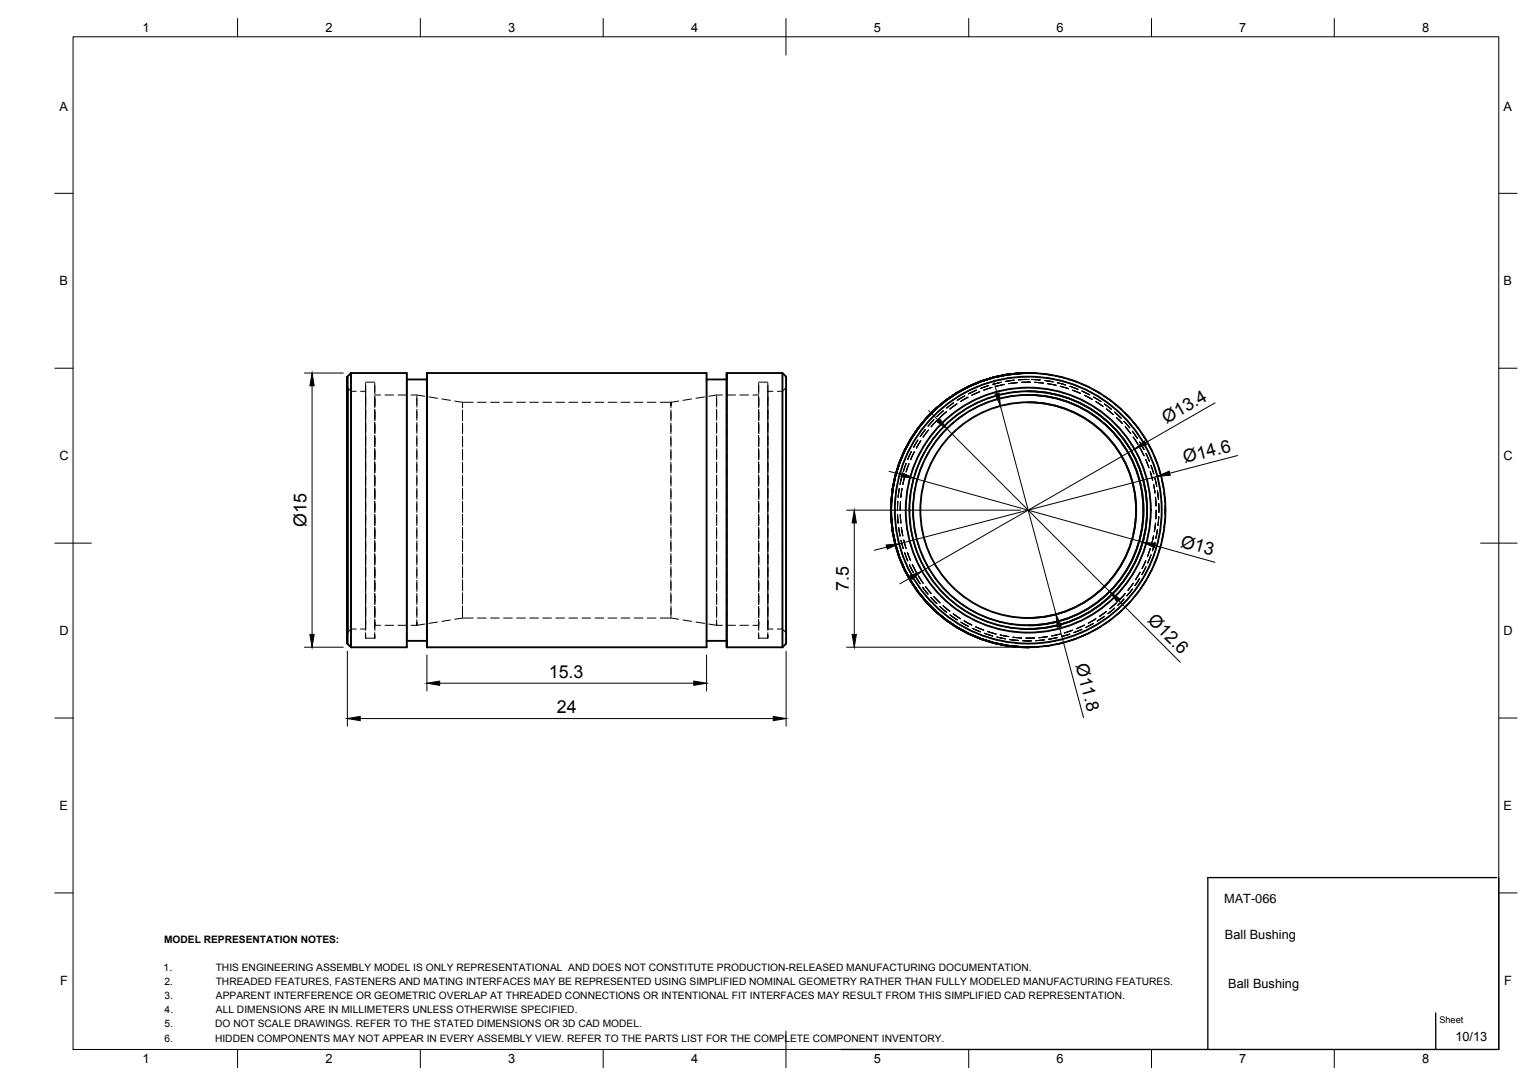
ISO-10303-21;
HEADER;
/* Generated by software containing ST-Developer
 * from STEP Tools, Inc. (www.steptools.com) 
 */

FILE_DESCRIPTION(
/* description */ ('CAx-IF Rec.Pracs.---Representation and Presentation of Product Manufa
cturing Information (PMI)---4.0---2014-10-13'),
/* implementation_level */ '2;1');

FILE_NAME(
/* name */ 'Ball Bushing.step',
/* time_stamp */ '2026-10-24T15:58:00-07:00',
/* author */ (''),
/* organization */ (''),
/* preprocessor_version */ 'ST-DEVELOPER v20.2',
/* originating_system */ 'Autodesk Translation Framework v15.17.0.0',
/* authorisation */ '');

FILE_SCHEMA (('AP242_MANAGED_MODEL_BASED_3D_ENGINEERING_MIM_LF { 1 0 10303 442 2 1 4 }'));
ENDSEC;

DATA;
#10=MECHANICAL_DESIGN_GEOMETRIC_PRESENTATION_REPRESENTATION('',(#134),#8944);
#99=CONICAL_SURFACE('',#5696,0.0066,0.785398163397459);
#100=CONICAL_SURFACE('',#5704,0.0074,0.785398163397448);
#101=CONICAL_SURFACE('',#5709,0.0066,0.785398163397459);
#102=CONICAL_SURFACE('',#5717,0.0074,0.785398163397448);
#103=CONICAL_SURFACE('',#5730,0.0061,0.158655262186402);
#104=CONICAL_SURFACE('',#5734,0.0061,0.158655262186402);
#116=SHAPE_REPRESENTATION_RELATIONSHIP('SRR','None',#8999,#125);
#125=ADVANCED_BREP_SHAPE_REPRESENTATION('',(#143),#8940);
#134=STYLED_ITEM('',(#9054),#143);
#143=MANIFOLD_SOLID_BREP('Body1',#5155);
#220=CYLINDRICAL_SURFACE('',#5702,0.0065);
#221=CYLINDRICAL_SURFACE('',#5707,0.0075);
#222=CYLINDRICAL_SURFACE('',#5715,0.0065);
#223=CYLINDRICAL_SURFACE('',#5720,0.0075);
#224=CYLINDRICAL_SURFACE('',#5724,0.00700000010430813);
#225=CYLINDRICAL_SURFACE('',#5728,0.0063);
#226=CYLINDRICAL_SURFACE('',#5732,0.0059);
#227=CYLINDRICAL_SURFACE('',#5736,0.0063);
#228=CYLINDRICAL_SURFACE('',#5740,0.00700000010430813);
#229=CYLINDRICAL_SURFACE('',#5745,0.00715);
#230=CYLINDRICAL_SURFACE('',#5749,0.0075);
#231=CYLINDRICAL_SURFACE('',#5753,0.00715);
#290=FACE_BOUND('',#854,.T.);
#291=FACE_BOUND('',#860,.T.);
#292=FACE_BOUND('',#865,.T.);
#293=FACE_BOUND('',#868,.T.);
#294=FACE_BOUND('',#875,.T.);
#295=FACE_BOUND('',#878,.T.);
#296=FACE_BOUND('',#880,.T.);
#297=FACE_BOUND('',#883,.T.);
#298=FACE_BOUND('',#886,.T.);
#299=FACE_BOUND('',#889,.T.);
#531=FACE_OUTER_BOUND('',#852,.T.);
#532=FACE_OUTER_BOUND('',#853,.T.);
#533=FACE_OUTER_BOUND('',#855,.T.);
#534=FACE_OUTER_BOUND('',#856,.T.);
#535=FACE_OUTER_BOUND('',#857,.T.);
#536=FACE_OUTER_BOUND('',#858,.T.);
#537=FACE_OUTER_BOUND('',#859,.T.);
#538=FACE_OUTER_BOUND('',#861,.T.);
#539=FACE_OUTER_BOUND('',#862,.T.);
#540=FACE_OUTER_BOUND('',#863,.T.);
#541=FACE_OUTER_BOUND('',#864,.T.);
#542=FACE_OUTER_BOUND('',#866,.T.);
#543=FACE_OUTER_BOUND('',#867,.T.);
#544=FACE_OUTER_BOUND('',#869,.T.);
#545=FACE_OUTER_BOUND('',#870,.T.);
#546=FACE_OUTER_BOUND('',#871,.T.);
#547=FACE_OUTER_BOUND('',#872,.T.);
#548=FACE_OUTER_BOUND('',#873,.T.);
#549=FACE_OUTER_BOUND('',#874,.T.);
#550=FACE_OUTER_BOUND('',#876,.T.);
#551=FACE_OUTER_BOUND('',#877,.T.);
#552=FACE_OUTER_BOUND('',#879,.T.);
#553=FACE_OUTER_BOUND('',#881,.T.);
#554=FACE_OUTER_BOUND('',#882,.T.);
#555=FACE_OUTER_BOUND('',#884,.T.);
#556=FACE_OUTER_BOUND('',#885,.T.);
#557=FACE_OUTER_BOUND('',#887,.T.);
#558=FACE_OUTER_BOUND('',#888,.T.);
#852=EDGE_LOOP('',(#4553,#4554,#4555,#4556,#4557));
#853=EDGE_LOOP('',(#4558));
#854=EDGE_LOOP('',(#4559));
#855=EDGE_LOOP('',(#4560,#4561,#4562,#4563,#4564));
#856=EDGE_LOOP('',(#4565,#4566,#4567,#4568,#4569));
#857=EDGE_LOOP('',(#4570,#4571,#4572,#4573,#4574));
#858=EDGE_LOOP('',(#4575,#4576,#4577,#4578,#4579));
#859=EDGE_LOOP('',(#4580));
#860=EDGE_LOOP('',(#4581));
#861=EDGE_LOOP('',(#4582,#4583,#4584,#4585,#4586));
#862=EDGE_LOOP('',(#4587,#4588,#4589,#4590,#4591));
#863=EDGE_LOOP('',(#4592,#4593,#4594,#4595,#4596));
#864=EDGE_LOOP('',(#4597));
#865=EDGE_LOOP('',(#4598));
#866=EDGE_LOOP('',(#4599,#4600,#4601,#4602));
#867=EDGE_LOOP('',(#4603));
#868=EDGE_LOOP('',(#4604));
#869=EDGE_LOOP('',(#4605,#4606,#4607,#4608));
#870=EDGE_LOOP('',(#4609,#4610,#4611,#4612));
#871=EDGE_LOOP('',(#4613,#4614,#4615,#4616));
#872=EDGE_LOOP('',(#4617,#4618,#4619,#4620));
#873=EDGE_LOOP('',(#4621,#4622,#4623,#4624));
#874=EDGE_LOOP('',(#4625));
#875=EDGE_LOOP('',(#4626));
#876=EDGE_LOOP('',(#4627,#4628,#4629,#4630));
#877=EDGE_LOOP('',(#4631));
#878=EDGE_LOOP('',(#4632));
#879=EDGE_LOOP('',(#4633));
#880=EDGE_LOOP('',(#4634));
#881=EDGE_LOOP('',(#4635,#4636,#4637,#4638));
#882=EDGE_LOOP('',(#4639));
#883=EDGE_LOOP('',(#4640));
#884=EDGE_LOOP('',(#4641,#4642,#4643,#4644));
#885=EDGE_LOOP('',(#4645));
#886=EDGE_LOOP('',(#4646));
#887=EDGE_LOOP('',(#4647,#4648,#4649,#4650));
#888=EDGE_LOOP('',(#4651));
#889=EDGE_LOOP('',(#4652));
#1122=CIRCLE('',#5697,0.00650000000001);
#1123=CIRCLE('',#5698,0.00670000000001);
#1124=CIRCLE('',#5699,0.00650000000001);
#1125=CIRCLE('',#5701,0.00730000000001);
#1126=CIRCLE('',#5703,0.00650000000001);
#1127=CIRCLE('',#5705,0.00750000000001);
#1128=CIRCLE('',#5706,0.00750000000001);
#1129=CIRCLE('',#5708,0.00750000000001);
#1130=CIRCLE('',#5710,0.00650000000001);
#1131=CIRCLE('',#5711,0.00670000000001);
#1132=CIRCLE('',#5712,0.00650000000001);
#1133=CIRCLE('',#5714,0.00730000000001);
#1134=CIRCLE('',#5716,0.00650000000001);
#1135=CIRCLE('',#5718,0.00750000000001);
#1136=CIRCLE('',#5719,0.00750000000001);
#1137=CIRCLE('',#5721,0.00750000000001);
#1138=CIRCLE('',#5723,0.00700000010431813);
#1139=CIRCLE('',#5725,0.00700000010431813);
#1140=CIRCLE('',#5727,0.00630000000001);
#1141=CIRCLE('',#5729,0.00630000000001);
#1142=CIRCLE('',#5731,0.00590000000001);
#1143=CIRCLE('',#5733,0.00590000000001);
#1144=CIRCLE('',#5735,0.00630000000001);
#1145=CIRCLE('',#5737,0.00630000000001);
#1146=CIRCLE('',#5739,0.00700000010431813);
#1147=CIRCLE('',#5741,0.00700000010431813);
#1148=CIRCLE('',#5744,0.00715000000001);
#1149=CIRCLE('',#5746,0.00715000000001);
#1150=CIRCLE('',#5748,0.00750000000001);
#1151=CIRCLE('',#5750,0.00750000000001);
#1152=CIRCLE('',#5752,0.00715000000001);
#1153=CIRCLE('',#5754,0.00715000000001);
#1599=LINE('',#8727,#2054);
#1600=LINE('',#8735,#2055);
#1601=LINE('',#8741,#2056);
#1602=LINE('',#8746,#2057);
#1603=LINE('',#8752,#2058);
#1604=LINE('',#8761,#2059);
#1605=LINE('',#8766,#2060);
#1606=LINE('',#8770,#2061);
#1607=LINE('',#8778,#2062);
#1608=LINE('',#8785,#2063);
#1609=LINE('',#8789,#2064);
#1610=LINE('',#8793,#2065);
#1611=LINE('',#8796,#2066);
#1612=LINE('',#8801,#2067);
#1613=LINE('',#8808,#2068);
#1614=LINE('',#8816,#2069);
#1615=LINE('',#8823,#2070);
#1616=LINE('',#8830,#2071);
#2054=VECTOR('',#7122,0.0066);
#2055=VECTOR('',#7133,0.0065);
#2056=VECTOR('',#7140,0.0074);
#2057=VECTOR('',#7147,0.0075);
#2058=VECTOR('',#7152,0.0066);
#2059=VECTOR('',#7165,0.0065);
#2060=VECTOR('',#7170,0.0074);
#2061=VECTOR('',#7175,0.0075);
#2062=VECTOR('',#7186,0.00700000010430813);
#2063=VECTOR('',#7195,0.0063);
#2064=VECTOR('',#7200,0.0061);
#2065=VECTOR('',#7205,0.0059);
#2066=VECTOR('',#7208,0.0061);
#2067=VECTOR('',#7215,0.0063);
#2068=VECTOR('',#7224,0.00700000010430813);
#2069=VECTOR('',#7235,0.00715);
#2070=VECTOR('',#7244,0.0075);
#2071=VECTOR('',#7253,0.00715);
#2508=VERTEX_POINT('',#8723);
#2509=VERTEX_POINT('',#8724);
#2510=VERTEX_POINT('',#8726);
#2511=VERTEX_POINT('',#8731);
#2512=VERTEX_POINT('',#8734);
#2513=VERTEX_POINT('',#8738);
#2514=VERTEX_POINT('',#8739);
#2515=VERTEX_POINT('',#8744);
#2516=VERTEX_POINT('',#8748);
#2517=VERTEX_POINT('',#8749);
#2518=VERTEX_POINT('',#8751);
#2519=VERTEX_POINT('',#8756);
#2520=VERTEX_POINT('',#8759);
#2521=VERTEX_POINT('',#8763);
#2522=VERTEX_POINT('',#8764);
#2523=VERTEX_POINT('',#8769);
#2524=VERTEX_POINT('',#8773);
#2525=VERTEX_POINT('',#8776);
#2526=VERTEX_POINT('',#8780);
#2527=VERTEX_POINT('',#8783);
#2528=VERTEX_POINT('',#8787);
#2529=VERTEX_POINT('',#8791);
#2530=VERTEX_POINT('',#8795);
#2531=VERTEX_POINT('',#8799);
#2532=VERTEX_POINT('',#8803);
#2533=VERTEX_POINT('',#8806);
#2534=VERTEX_POINT('',#8811);
#2535=VERTEX_POINT('',#8814);
#2536=VERTEX_POINT('',#8818);
#2537=VERTEX_POINT('',#8821);
#2538=VERTEX_POINT('',#8825);
#2539=VERTEX_POINT('',#8828);
#3197=EDGE_CURVE('',#2508,#2509,#1122,.T.);
#3198=EDGE_CURVE('',#2509,#2510,#1599,.T.);
#3199=EDGE_CURVE('',#2510,#2510,#1123,.T.);
#3200=EDGE_CURVE('',#2509,#2508,#1124,.T.);
#3201=EDGE_CURVE('',#2511,#2511,#1125,.T.);
#3202=EDGE_CURVE('',#2508,#2512,#1600,.T.);
#3203=EDGE_CURVE('',#2512,#2512,#1126,.T.);
#3204=EDGE_CURVE('',#2513,#2514,#1127,.T.);
#3205=EDGE_CURVE('',#2514,#2511,#1601,.T.);
#3206=EDGE_CURVE('',#2514,#2513,#1128,.T.);
#3207=EDGE_CURVE('',#2515,#2515,#1129,.T.);
#3208=EDGE_CURVE('',#2515,#2513,#1602,.T.);
#3209=EDGE_CURVE('',#2516,#2517,#1130,.T.);
#3210=EDGE_CURVE('',#2517,#2518,#1603,.T.);
#3211=EDGE_CURVE('',#2518,#2518,#1131,.T.);
#3212=EDGE_CURVE('',#2517,#2516,#1132,.T.);
#3213=EDGE_CURVE('',#2519,#2519,#1133,.T.);
#3214=EDGE_CURVE('',#2520,#2520,#1134,.T.);
#3215=EDGE_CURVE('',#2520,#2516,#1604,.T.);
#3216=EDGE_CURVE('',#2521,#2522,#1135,.T.);
#3217=EDGE_CURVE('',#2522,#2519,#1605,.T.);
#3218=EDGE_CURVE('',#2522,#2521,#1136,.T.);
#3219=EDGE_CURVE('',#2521,#2523,#1606,.T.);
#3220=EDGE_CURVE('',#2523,#2523,#1137,.T.);
#3221=EDGE_CURVE('',#2524,#2524,#1138,.T.);
#3222=EDGE_CURVE('',#2525,#2525,#1139,.T.);
#3223=EDGE_CURVE('',#2525,#2524,#1607,.T.);
#3224=EDGE_CURVE('',#2526,#2526,#1140,.T.);
#3225=EDGE_CURVE('',#2527,#2527,#1141,.T.);
#3226=EDGE_CURVE('',#2527,#2526,#1608,.T.);
#3227=EDGE_CURVE('',#2528,#2528,#1142,.T.);
#3228=EDGE_CURVE('',#2528,#2527,#1609,.T.);
#3229=EDGE_CURVE('',#2529,#2529,#1143,.T.);
#3230=EDGE_CURVE('',#2529,#2528,#1610,.T.);
#3231=EDGE_CURVE('',#2529,#2530,#1611,.T.);
#3232=EDGE_CURVE('',#2530,#2530,#1144,.T.);
#3233=EDGE_CURVE('',#2531,#2531,#1145,.T.);
#3234=EDGE_CURVE('',#2531,#2530,#1612,.T.);
#3235=EDGE_CURVE('',#2532,#2532,#1146,.T.);
#3236=EDGE_CURVE('',#2533,#2533,#1147,.T.);
#3237=EDGE_CURVE('',#2533,#2532,#1613,.T.);
#3238=EDGE_CURVE('',#2534,#2534,#1148,.T.);
#3239=EDGE_CURVE('',#2535,#2535,#1149,.T.);
#3240=EDGE_CURVE('',#2535,#2534,#1614,.T.);
#3241=EDGE_CURVE('',#2536,#2536,#1150,.T.);
#3242=EDGE_CURVE('',#2537,#2537,#1151,.T.);
#3243=EDGE_CURVE('',#2537,#2536,#1615,.T.);
#3244=EDGE_CURVE('',#2538,#2538,#1152,.T.);
#3245=EDGE_CURVE('',#2539,#2539,#1153,.T.);
#3246=EDGE_CURVE('',#2539,#2538,#1616,.T.);
#4553=ORIENTED_EDGE('',*,*,#3197,.T.);
#4554=ORIENTED_EDGE('',*,*,#3198,.T.);
#4555=ORIENTED_EDGE('',*,*,#3199,.T.);
#4556=ORIENTED_EDGE('',*,*,#3198,.F.);
#4557=ORIENTED_EDGE('',*,*,#3200,.T.);
#4558=ORIENTED_EDGE('',*,*,#3201,.F.);
#4559=ORIENTED_EDGE('',*,*,#3199,.F.);
#4560=ORIENTED_EDGE('',*,*,#3197,.F.);
#4561=ORIENTED_EDGE('',*,*,#3202,.T.);
#4562=ORIENTED_EDGE('',*,*,#3203,.T.);
#4563=ORIENTED_EDGE('',*,*,#3202,.F.);
#4564=ORIENTED_EDGE('',*,*,#3200,.F.);
#4565=ORIENTED_EDGE('',*,*,#3204,.T.);
#4566=ORIENTED_EDGE('',*,*,#3205,.T.);
#4567=ORIENTED_EDGE('',*,*,#3201,.T.);
#4568=ORIENTED_EDGE('',*,*,#3205,.F.);
#4569=ORIENTED_EDGE('',*,*,#3206,.T.);
#4570=ORIENTED_EDGE('',*,*,#3207,.F.);
#4571=ORIENTED_EDGE('',*,*,#3208,.T.);
#4572=ORIENTED_EDGE('',*,*,#3206,.F.);
#4573=ORIENTED_EDGE('',*,*,#3204,.F.);
#4574=ORIENTED_EDGE('',*,*,#3208,.F.);
#4575=ORIENTED_EDGE('',*,*,#3209,.T.);
#4576=ORIENTED_EDGE('',*,*,#3210,.T.);
#4577=ORIENTED_EDGE('',*,*,#3211,.T.);
#4578=ORIENTED_EDGE('',*,*,#3210,.F.);
#4579=ORIENTED_EDGE('',*,*,#3212,.T.);
#4580=ORIENTED_EDGE('',*,*,#3213,.F.);
#4581=ORIENTED_EDGE('',*,*,#3211,.F.);
#4582=ORIENTED_EDGE('',*,*,#3214,.F.);
#4583=ORIENTED_EDGE('',*,*,#3215,.T.);
#4584=ORIENTED_EDGE('',*,*,#3212,.F.);
#4585=ORIENTED_EDGE('',*,*,#3209,.F.);
#4586=ORIENTED_EDGE('',*,*,#3215,.F.);
#4587=ORIENTED_EDGE('',*,*,#3216,.T.);
#4588=ORIENTED_EDGE('',*,*,#3217,.T.);
#4589=ORIENTED_EDGE('',*,*,#3213,.T.);
#4590=ORIENTED_EDGE('',*,*,#3217,.F.);
#4591=ORIENTED_EDGE('',*,*,#3218,.T.);
#4592=ORIENTED_EDGE('',*,*,#3216,.F.);
#4593=ORIENTED_EDGE('',*,*,#3219,.T.);
#4594=ORIENTED_EDGE('',*,*,#3220,.T.);
#4595=ORIENTED_EDGE('',*,*,#3219,.F.);
#4596=ORIENTED_EDGE('',*,*,#3218,.F.);
#4597=ORIENTED_EDGE('',*,*,#3221,.F.);
#4598=ORIENTED_EDGE('',*,*,#3214,.T.);
#4599=ORIENTED_EDGE('',*,*,#3222,.F.);
#4600=ORIENTED_EDGE('',*,*,#3223,.T.);
#4601=ORIENTED_EDGE('',*,*,#3221,.T.);
#4602=ORIENTED_EDGE('',*,*,#3223,.F.);
#4603=ORIENTED_EDGE('',*,*,#3222,.T.);
#4604=ORIENTED_EDGE('',*,*,#3224,.F.);
#4605=ORIENTED_EDGE('',*,*,#3225,.F.);
#4606=ORIENTED_EDGE('',*,*,#3226,.T.);
#4607=ORIENTED_EDGE('',*,*,#3224,.T.);
#4608=ORIENTED_EDGE('',*,*,#3226,.F.);
#4609=ORIENTED_EDGE('',*,*,#3227,.F.);
#4610=ORIENTED_EDGE('',*,*,#3228,.T.);
#4611=ORIENTED_EDGE('',*,*,#3225,.T.);
#4612=ORIENTED_EDGE('',*,*,#3228,.F.);
#4613=ORIENTED_EDGE('',*,*,#3229,.F.);
#4614=ORIENTED_EDGE('',*,*,#3230,.T.);
#4615=ORIENTED_EDGE('',*,*,#3227,.T.);
#4616=ORIENTED_EDGE('',*,*,#3230,.F.);
#4617=ORIENTED_EDGE('',*,*,#3229,.T.);
#4618=ORIENTED_EDGE('',*,*,#3231,.T.);
#4619=ORIENTED_EDGE('',*,*,#3232,.F.);
#4620=ORIENTED_EDGE('',*,*,#3231,.F.);
#4621=ORIENTED_EDGE('',*,*,#3233,.F.);
#4622=ORIENTED_EDGE('',*,*,#3234,.T.);
#4623=ORIENTED_EDGE('',*,*,#3232,.T.);
#4624=ORIENTED_EDGE('',*,*,#3234,.F.);
#4625=ORIENTED_EDGE('',*,*,#3235,.F.);
#4626=ORIENTED_EDGE('',*,*,#3233,.T.);
#4627=ORIENTED_EDGE('',*,*,#3236,.F.);
#4628=ORIENTED_EDGE('',*,*,#3237,.T.);
#4629=ORIENTED_EDGE('',*,*,#3235,.T.);
#4630=ORIENTED_EDGE('',*,*,#3237,.F.);
#4631=ORIENTED_EDGE('',*,*,#3236,.T.);
#4632=ORIENTED_EDGE('',*,*,#3203,.F.);
#4633=ORIENTED_EDGE('',*,*,#3207,.T.);
#4634=ORIENTED_EDGE('',*,*,#3238,.F.);
#4635=ORIENTED_EDGE('',*,*,#3239,.F.);
#4636=ORIENTED_EDGE('',*,*,#3240,.T.);
#4637=ORIENTED_EDGE('',*,*,#3238,.T.);
#4638=ORIENTED_EDGE('',*,*,#3240,.F.);
#4639=ORIENTED_EDGE('',*,*,#3241,.F.);
#4640=ORIENTED_EDGE('',*,*,#3239,.T.);
#4641=ORIENTED_EDGE('',*,*,#3242,.F.);
#4642=ORIENTED_EDGE('',*,*,#3243,.T.);
#4643=ORIENTED_EDGE('',*,*,#3241,.T.);
#4644=ORIENTED_EDGE('',*,*,#3243,.F.);
#4645=ORIENTED_EDGE('',*,*,#3242,.T.);
#4646=ORIENTED_EDGE('',*,*,#3244,.F.);
#4647=ORIENTED_EDGE('',*,*,#3245,.F.);
#4648=ORIENTED_EDGE('',*,*,#3246,.T.);
#4649=ORIENTED_EDGE('',*,*,#3244,.T.);
#4650=ORIENTED_EDGE('',*,*,#3246,.F.);
#4651=ORIENTED_EDGE('',*,*,#3220,.F.);
#4652=ORIENTED_EDGE('',*,*,#3245,.T.);
#4863=PLANE('',#5700);
#4864=PLANE('',#5713);
#4865=PLANE('',#5722);
#4866=PLANE('',#5726);
#4867=PLANE('',#5738);
#4868=PLANE('',#5742);
#4869=PLANE('',#5743);
#4870=PLANE('',#5747);
#4871=PLANE('',#5751);
#4872=PLANE('',#5755);
#5104=ADVANCED_FACE('',(#531),#99,.F.);
#5105=ADVANCED_FACE('',(#532,#290),#4863,.T.);
#5106=ADVANCED_FACE('',(#533),#220,.F.);
#5107=ADVANCED_FACE('',(#534),#100,.T.);
#5108=ADVANCED_FACE('',(#535),#221,.T.);
#5109=ADVANCED_FACE('',(#536),#101,.F.);
#5110=ADVANCED_FACE('',(#537,#291),#4864,.T.);
#5111=ADVANCED_FACE('',(#538),#222,.F.);
#5112=ADVANCED_FACE('',(#539),#102,.T.);
#5113=ADVANCED_FACE('',(#540),#223,.T.);
#5114=ADVANCED_FACE('',(#541,#292),#4865,.T.);
#5115=ADVANCED_FACE('',(#542),#224,.F.);
#5116=ADVANCED_FACE('',(#543,#293),#4866,.T.);
#5117=ADVANCED_FACE('',(#544),#225,.F.);
#5118=ADVANCED_FACE('',(#545),#103,.F.);
#5119=ADVANCED_FACE('',(#546),#226,.F.);
#5120=ADVANCED_FACE('',(#547),#104,.F.);
#5121=ADVANCED_FACE('',(#548),#227,.F.);
#5122=ADVANCED_FACE('',(#549,#294),#4867,.T.);
#5123=ADVANCED_FACE('',(#550),#228,.F.);
#5124=ADVANCED_FACE('',(#551,#295),#4868,.T.);
#5125=ADVANCED_FACE('',(#552,#296),#4869,.T.);
#5126=ADVANCED_FACE('',(#553),#229,.T.);
#5127=ADVANCED_FACE('',(#554,#297),#4870,.T.);
#5128=ADVANCED_FACE('',(#555),#230,.T.);
#5129=ADVANCED_FACE('',(#556,#298),#4871,.T.);
#5130=ADVANCED_FACE('',(#557),#231,.T.);
#5131=ADVANCED_FACE('',(#558,#299),#4872,.T.);
#5155=CLOSED_SHELL('',(#5104,#5105,#5106,#5107,#5108,#5109,#5110,#5111,
#5112,#5113,#5114,#5115,#5116,#5117,#5118,#5119,#5120,#5121,#5122,#5123,
#5124,#5125,#5126,#5127,#5128,#5129,#5130,#5131));
#5695=AXIS2_PLACEMENT_3D('',#8721,#7116,#7117);
#5696=AXIS2_PLACEMENT_3D('',#8722,#7118,#7119);
#5697=AXIS2_PLACEMENT_3D('',#8725,#7120,#7121);
#5698=AXIS2_PLACEMENT_3D('',#8728,#7123,#7124);
#5699=AXIS2_PLACEMENT_3D('',#8729,#7125,#7126);
#5700=AXIS2_PLACEMENT_3D('',#8730,#7127,#7128);
#5701=AXIS2_PLACEMENT_3D('',#8732,#7129,#7130);
#5702=AXIS2_PLACEMENT_3D('',#8733,#7131,#7132);
#5703=AXIS2_PLACEMENT_3D('',#8736,#7134,#7135);
#5704=AXIS2_PLACEMENT_3D('',#8737,#7136,#7137);
#5705=AXIS2_PLACEMENT_3D('',#8740,#7138,#7139);
#5706=AXIS2_PLACEMENT_3D('',#8742,#7141,#7142);
#5707=AXIS2_PLACEMENT_3D('',#8743,#7143,#7144);
#5708=AXIS2_PLACEMENT_3D('',#8745,#7145,#7146);
#5709=AXIS2_PLACEMENT_3D('',#8747,#7148,#7149);
#5710=AXIS2_PLACEMENT_3D('',#8750,#7150,#7151);
#5711=AXIS2_PLACEMENT_3D('',#8753,#7153,#7154);
#5712=AXIS2_PLACEMENT_3D('',#8754,#7155,#7156);
#5713=AXIS2_PLACEMENT_3D('',#8755,#7157,#7158);
#5714=AXIS2_PLACEMENT_3D('',#8757,#7159,#7160);
#5715=AXIS2_PLACEMENT_3D('',#8758,#7161,#7162);
#5716=AXIS2_PLACEMENT_3D('',#8760,#7163,#7164);
#5717=AXIS2_PLACEMENT_3D('',#8762,#7166,#7167);
#5718=AXIS2_PLACEMENT_3D('',#8765,#7168,#7169);
#5719=AXIS2_PLACEMENT_3D('',#8767,#7171,#7172);
#5720=AXIS2_PLACEMENT_3D('',#8768,#7173,#7174);
#5721=AXIS2_PLACEMENT_3D('',#8771,#7176,#7177);
#5722=AXIS2_PLACEMENT_3D('',#8772,#7178,#7179);
#5723=AXIS2_PLACEMENT_3D('',#8774,#7180,#7181);
#5724=AXIS2_PLACEMENT_3D('',#8775,#7182,#7183);
#5725=AXIS2_PLACEMENT_3D('',#8777,#7184,#7185);
#5726=AXIS2_PLACEMENT_3D('',#8779,#7187,#7188);
#5727=AXIS2_PLACEMENT_3D('',#8781,#7189,#7190);
#5728=AXIS2_PLACEMENT_3D('',#8782,#7191,#7192);
#5729=AXIS2_PLACEMENT_3D('',#8784,#7193,#7194);
#5730=AXIS2_PLACEMENT_3D('',#8786,#7196,#7197);
#5731=AXIS2_PLACEMENT_3D('',#8788,#7198,#7199);
#5732=AXIS2_PLACEMENT_3D('',#8790,#7201,#7202);
#5733=AXIS2_PLACEMENT_3D('',#8792,#7203,#7204);
#5734=AXIS2_PLACEMENT_3D('',#8794,#7206,#7207);
#5735=AXIS2_PLACEMENT_3D('',#8797,#7209,#7210);
#5736=AXIS2_PLACEMENT_3D('',#8798,#7211,#7212);
#5737=AXIS2_PLACEMENT_3D('',#8800,#7213,#7214);
#5738=AXIS2_PLACEMENT_3D('',#8802,#7216,#7217);
#5739=AXIS2_PLACEMENT_3D('',#8804,#7218,#7219);
#5740=AXIS2_PLACEMENT_3D('',#8805,#7220,#7221);
#5741=AXIS2_PLACEMENT_3D('',#8807,#7222,#7223);
#5742=AXIS2_PLACEMENT_3D('',#8809,#7225,#7226);
#5743=AXIS2_PLACEMENT_3D('',#8810,#7227,#7228);
#5744=AXIS2_PLACEMENT_3D('',#8812,#7229,#7230);
#5745=AXIS2_PLACEMENT_3D('',#8813,#7231,#7232);
#5746=AXIS2_PLACEMENT_3D('',#8815,#7233,#7234);
#5747=AXIS2_PLACEMENT_3D('',#8817,#7236,#7237);
#5748=AXIS2_PLACEMENT_3D('',#8819,#7238,#7239);
#5749=AXIS2_PLACEMENT_3D('',#8820,#7240,#7241);
#5750=AXIS2_PLACEMENT_3D('',#8822,#7242,#7243);
#5751=AXIS2_PLACEMENT_3D('',#8824,#7245,#7246);
#5752=AXIS2_PLACEMENT_3D('',#8826,#7247,#7248);
#5753=AXIS2_PLACEMENT_3D('',#8827,#7249,#7250);
#5754=AXIS2_PLACEMENT_3D('',#8829,#7251,#7252);
#5755=AXIS2_PLACEMENT_3D('',#8831,#7254,#7255);
#7116=DIRECTION('axis',(0.,0.,1.));
#7117=DIRECTION('refdir',(1.,0.,0.));
#7118=DIRECTION('center_axis',(0.,-1.,0.));
#7119=DIRECTION('ref_axis',(0.,0.,-1.));
#7120=DIRECTION('center_axis',(0.,1.,0.));
#7121=DIRECTION('ref_axis',(0.,0.,-1.));
#7122=DIRECTION('',(-8.65956056235503E-17,-0.70710678118654,0.707106781186555));
#7123=DIRECTION('center_axis',(0.,-1.,0.));
#7124=DIRECTION('ref_axis',(0.,0.,-1.));
#7125=DIRECTION('center_axis',(0.,1.,0.));
#7126=DIRECTION('ref_axis',(0.,0.,-1.));
#7127=DIRECTION('center_axis',(0.,-1.,0.));
#7128=DIRECTION('ref_axis',(0.,0.,-1.));
#7129=DIRECTION('center_axis',(0.,1.,0.));
#7130=DIRECTION('ref_axis',(0.,0.,-1.));
#7131=DIRECTION('center_axis',(0.,1.,0.));
#7132=DIRECTION('ref_axis',(0.,0.,1.));
#7133=DIRECTION('',(0.,1.,0.));
#7134=DIRECTION('center_axis',(0.,1.,0.));
#7135=DIRECTION('ref_axis',(1.,0.,0.));
#7136=DIRECTION('center_axis',(0.,1.,0.));
#7137=DIRECTION('ref_axis',(0.,0.,-1.));
#7138=DIRECTION('center_axis',(0.,-1.,0.));
#7139=DIRECTION('ref_axis',(0.,0.,-1.));
#7140=DIRECTION('',(-8.65956056235493E-17,-0.707106781186548,-0.707106781186547));
#7141=DIRECTION('center_axis',(0.,-1.,0.));
#7142=DIRECTION('ref_axis',(0.,0.,-1.));
#7143=DIRECTION('center_axis',(0.,1.,0.));
#7144=DIRECTION('ref_axis',(0.,0.,1.));
#7145=DIRECTION('center_axis',(0.,1.,0.));
#7146=DIRECTION('ref_axis',(1.,0.,0.));
#7147=DIRECTION('',(0.,-1.,0.));
#7148=DIRECTION('center_axis',(0.,1.,0.));
#7149=DIRECTION('ref_axis',(0.,0.,-1.));
#7150=DIRECTION('center_axis',(0.,-1.,0.));
#7151=DIRECTION('ref_axis',(0.,0.,-1.));
#7152=DIRECTION('',(8.65956056235503E-17,0.70710678118654,0.707106781186555));
#7153=DIRECTION('center_axis',(0.,1.,0.));
#7154=DIRECTION('ref_axis',(0.,0.,-1.));
#7155=DIRECTION('center_axis',(0.,-1.,0.));
#7156=DIRECTION('ref_axis',(0.,0.,-1.));
#7157=DIRECTION('center_axis',(0.,1.,0.));
#7158=DIRECTION('ref_axis',(1.,0.,0.));
#7159=DIRECTION('center_axis',(0.,-1.,0.));
#7160=DIRECTION('ref_axis',(0.,0.,-1.));
#7161=DIRECTION('center_axis',(0.,1.,0.));
#7162=DIRECTION('ref_axis',(0.,0.,1.));
#7163=DIRECTION('center_axis',(0.,1.,0.));
#7164=DIRECTION('ref_axis',(1.,0.,0.));
#7165=DIRECTION('',(0.,1.,0.));
#7166=DIRECTION('center_axis',(0.,-1.,0.));
#7167=DIRECTION('ref_axis',(0.,0.,-1.));
#7168=DIRECTION('center_axis',(0.,1.,0.));
#7169=DIRECTION('ref_axis',(0.,0.,-1.));
#7170=DIRECTION('',(8.65956056235493E-17,0.707106781186548,-0.707106781186547));
#7171=DIRECTION('center_axis',(0.,1.,0.));
#7172=DIRECTION('ref_axis',(0.,0.,-1.));
#7173=DIRECTION('center_axis',(0.,1.,0.));
#7174=DIRECTION('ref_axis',(0.,0.,1.));
#7175=DIRECTION('',(0.,-1.,0.));
#7176=DIRECTION('center_axis',(0.,1.,0.));
#7177=DIRECTION('ref_axis',(1.,0.,0.));
#7178=DIRECTION('center_axis',(0.,-1.,0.));
#7179=DIRECTION('ref_axis',(0.,0.,-1.));
#7180=DIRECTION('center_axis',(0.,1.,0.));
#7181=DIRECTION('ref_axis',(1.,0.,0.));
#7182=DIRECTION('center_axis',(0.,1.,0.));
#7183=DIRECTION('ref_axis',(0.,0.,1.));
#7184=DIRECTION('center_axis',(0.,1.,0.));
#7185=DIRECTION('ref_axis',(1.,0.,0.));
#7186=DIRECTION('',(0.,1.,0.));
#7187=DIRECTION('center_axis',(0.,1.,0.));
#7188=DIRECTION('ref_axis',(1.,0.,0.));
#7189=DIRECTION('center_axis',(0.,1.,0.));
#7190=DIRECTION('ref_axis',(1.,0.,0.));
#7191=DIRECTION('center_axis',(0.,1.,0.));
#7192=DIRECTION('ref_axis',(0.,0.,1.));
#7193=DIRECTION('center_axis',(0.,1.,0.));
#7194=DIRECTION('ref_axis',(1.,0.,0.));
#7195=DIRECTION('',(0.,1.,0.));
#7196=DIRECTION('center_axis',(0.,1.,0.));
#7197=DIRECTION('ref_axis',(0.,0.,1.));
#7198=DIRECTION('center_axis',(0.,1.,0.));
#7199=DIRECTION('ref_axis',(1.,0.,0.));
#7200=DIRECTION('',(-1.93482561475974E-17,0.987440631916705,-0.157990501106673));
#7201=DIRECTION('center_axis',(0.,1.,0.));
#7202=DIRECTION('ref_axis',(0.,0.,1.));
#7203=DIRECTION('center_axis',(0.,1.,0.));
#7204=DIRECTION('ref_axis',(1.,0.,0.));
#7205=DIRECTION('',(0.,1.,0.));
#7206=DIRECTION('center_axis',(0.,-1.,0.));
#7207=DIRECTION('ref_axis',(0.,0.,1.));
#7208=DIRECTION('',(1.93482561475974E-17,-0.987440631916705,-0.157990501106673));
#7209=DIRECTION('center_axis',(0.,1.,0.));
#7210=DIRECTION('ref_axis',(1.,0.,0.));
#7211=DIRECTION('center_axis',(0.,1.,0.));
#7212=DIRECTION('ref_axis',(0.,0.,1.));
#7213=DIRECTION('center_axis',(0.,1.,0.));
#7214=DIRECTION('ref_axis',(1.,0.,0.));
#7215=DIRECTION('',(0.,1.,0.));
#7216=DIRECTION('center_axis',(0.,-1.,0.));
#7217=DIRECTION('ref_axis',(0.,0.,-1.));
#7218=DIRECTION('center_axis',(0.,1.,0.));
#7219=DIRECTION('ref_axis',(1.,0.,0.));
#7220=DIRECTION('center_axis',(0.,1.,0.));
#7221=DIRECTION('ref_axis',(0.,0.,1.));
#7222=DIRECTION('center_axis',(0.,1.,0.));
#7223=DIRECTION('ref_axis',(1.,0.,0.));
#7224=DIRECTION('',(0.,1.,0.));
#7225=DIRECTION('center_axis',(0.,1.,0.));
#7226=DIRECTION('ref_axis',(1.,0.,0.));
#7227=DIRECTION('center_axis',(0.,1.,0.));
#7228=DIRECTION('ref_axis',(1.,0.,0.));
#7229=DIRECTION('center_axis',(0.,1.,0.));
#7230=DIRECTION('ref_axis',(1.,0.,0.));
#7231=DIRECTION('center_axis',(0.,1.,0.));
#7232=DIRECTION('ref_axis',(0.,0.,1.));
#7233=DIRECTION('center_axis',(0.,1.,0.));
#7234=DIRECTION('ref_axis',(1.,0.,0.));
#7235=DIRECTION('',(0.,-1.,0.));
#7236=DIRECTION('center_axis',(0.,-1.,0.));
#7237=DIRECTION('ref_axis',(0.,0.,-1.));
#7238=DIRECTION('center_axis',(0.,1.,0.));
#7239=DIRECTION('ref_axis',(1.,0.,0.));
#7240=DIRECTION('center_axis',(0.,1.,0.));
#7241=DIRECTION('ref_axis',(0.,0.,1.));
#7242=DIRECTION('center_axis',(0.,1.,0.));
#7243=DIRECTION('ref_axis',(1.,0.,0.));
#7244=DIRECTION('',(0.,-1.,0.));
#7245=DIRECTION('center_axis',(0.,1.,0.));
#7246=DIRECTION('ref_axis',(1.,0.,0.));
#7247=DIRECTION('center_axis',(0.,1.,0.));
#7248=DIRECTION('ref_axis',(1.,0.,0.));
#7249=DIRECTION('center_axis',(0.,1.,0.));
#7250=DIRECTION('ref_axis',(0.,0.,1.));
#7251=DIRECTION('center_axis',(0.,1.,0.));
#7252=DIRECTION('ref_axis',(1.,0.,0.));
#7253=DIRECTION('',(0.,-1.,0.));
#7254=DIRECTION('center_axis',(0.,-1.,0.));
#7255=DIRECTION('ref_axis',(0.,0.,-1.));
#8721=CARTESIAN_POINT('',(0.,0.,0.));
#8722=CARTESIAN_POINT('Origin',(0.,-0.0119,0.));
#8723=CARTESIAN_POINT('',(0.,-0.01180000000001,-0.00650000000001));
#8724=CARTESIAN_POINT('',(-7.96020419447004E-19,-0.01180000000001,0.00650000000001));
#8725=CARTESIAN_POINT('Origin',(0.,-0.01180000000001,0.));
#8726=CARTESIAN_POINT('',(-8.20513355429951E-19,-0.01200000000001,0.00670000000001));
#8727=CARTESIAN_POINT('',(-8.08266887437253E-19,-0.0119,0.0066));
#8728=CARTESIAN_POINT('Origin',(0.,-0.01200000000001,0.));
#8729=CARTESIAN_POINT('Origin',(0.,-0.01180000000001,0.));
#8730=CARTESIAN_POINT('Origin',(0.,-0.012,0.0075));
#8731=CARTESIAN_POINT('',(8.93992163377568E-19,-0.012,0.0073));
#8732=CARTESIAN_POINT('Origin',(0.,-0.01200000000001,0.));
#8733=CARTESIAN_POINT('Origin',(0.,-0.0115000000819564,0.));
#8734=CARTESIAN_POINT('',(-7.9602041944578E-19,-0.0110000001639228,-0.0065));
#8735=CARTESIAN_POINT('',(-7.9602041944578E-19,-0.0115000000819564,-0.0065));
#8736=CARTESIAN_POINT('Origin',(0.,-0.0110000001639228,0.));
#8737=CARTESIAN_POINT('Origin',(0.,-0.0119,0.));
#8738=CARTESIAN_POINT('',(0.,-0.01180000000001,-0.00750000000001));
#8739=CARTESIAN_POINT('',(9.18485099360515E-19,-0.0118,0.0075));
#8740=CARTESIAN_POINT('Origin',(0.,-0.01180000000001,0.));
#8741=CARTESIAN_POINT('',(9.06238631369041E-19,-0.0119,0.0074));
#8742=CARTESIAN_POINT('Origin',(0.,-0.01180000000001,0.));
#8743=CARTESIAN_POINT('Origin',(0.,-0.010375,0.));
#8744=CARTESIAN_POINT('',(-9.18485099360515E-19,-0.00875000000001,-0.0075));
#8745=CARTESIAN_POINT('Origin',(0.,-0.00875000000001,0.));
#8746=CARTESIAN_POINT('',(-9.18485099360515E-19,-0.010375,-0.0075));
#8747=CARTESIAN_POINT('Origin',(0.,0.0119,0.));
#8748=CARTESIAN_POINT('',(0.,0.01180000000001,-0.00650000000001));
#8749=CARTESIAN_POINT('',(7.96020419447004E-19,0.01180000000001,0.00650000000001));
#8750=CARTESIAN_POINT('Origin',(0.,0.01180000000001,0.));
#8751=CARTESIAN_POINT('',(8.20513355429951E-19,0.01200000000001,0.00670000000001));
#8752=CARTESIAN_POINT('',(8.08266887437253E-19,0.0119,0.0066));
#8753=CARTESIAN_POINT('Origin',(0.,0.01200000000001,0.));
#8754=CARTESIAN_POINT('Origin',(0.,0.01180000000001,0.));
#8755=CARTESIAN_POINT('Origin',(0.,0.012,0.0065));
#8756=CARTESIAN_POINT('',(-8.93992163377568E-19,0.012,0.0073));
#8757=CARTESIAN_POINT('Origin',(0.,0.01200000000001,0.));
#8758=CARTESIAN_POINT('Origin',(0.,0.0115000000819564,0.));
#8759=CARTESIAN_POINT('',(-7.9602041944578E-19,0.0110000001639228,-0.0065));
#8760=CARTESIAN_POINT('Origin',(0.,0.0110000001639228,0.));
#8761=CARTESIAN_POINT('',(-7.9602041944578E-19,0.0115000000819564,-0.0065));
#8762=CARTESIAN_POINT('Origin',(0.,0.0119,0.));
#8763=CARTESIAN_POINT('',(0.,0.01180000000001,-0.00750000000001));
#8764=CARTESIAN_POINT('',(-9.18485099360515E-19,0.0118,0.0075));
#8765=CARTESIAN_POINT('Origin',(0.,0.01180000000001,0.));
#8766=CARTESIAN_POINT('',(-9.06238631369041E-19,0.0119,0.0074));
#8767=CARTESIAN_POINT('Origin',(0.,0.01180000000001,0.));
#8768=CARTESIAN_POINT('Origin',(0.,0.010375,0.));
#8769=CARTESIAN_POINT('',(-9.18485099360515E-19,0.00875000000001,-0.0075));
#8770=CARTESIAN_POINT('',(-9.18485099360515E-19,0.010375,-0.0075));
#8771=CARTESIAN_POINT('Origin',(0.,0.00875000000001,0.));
#8772=CARTESIAN_POINT('Origin',(0.,0.0110000001639128,0.00700000010430813));
#8773=CARTESIAN_POINT('',(-8.57252772177209E-19,0.0110000001639228,-0.00700000010430813));
#8774=CARTESIAN_POINT('Origin',(0.,0.0110000001639228,0.));
#8775=CARTESIAN_POINT('Origin',(0.,0.0107500001601875,0.));
#8776=CARTESIAN_POINT('',(-8.57252772177209E-19,0.0105000001564722,-0.00700000010430813));
#8777=CARTESIAN_POINT('Origin',(0.,0.0105000001564722,0.));
#8778=CARTESIAN_POINT('',(-8.57252772177209E-19,0.0107500001601875,-0.00700000010430813));
#8779=CARTESIAN_POINT('Origin',(0.,0.0105000001564622,0.0063));
#8780=CARTESIAN_POINT('',(-7.71527483462833E-19,0.0105000001564722,-0.0063));
#8781=CARTESIAN_POINT('Origin',(0.,0.0105000001564722,0.));
#8782=CARTESIAN_POINT('Origin',(0.,0.0093500000782311,0.));
#8783=CARTESIAN_POINT('',(-7.71527483462833E-19,0.00820000000001,-0.0063));
#8784=CARTESIAN_POINT('Origin',(0.,0.00820000000001,0.));
#8785=CARTESIAN_POINT('',(-7.71527483462833E-19,0.0093500000782311,-0.0063));
#8786=CARTESIAN_POINT('Origin',(0.,0.00695,0.));
#8787=CARTESIAN_POINT('',(-7.2254161149716E-19,0.00570000000001131,-0.00590000000000181));
#8788=CARTESIAN_POINT('Origin',(0.,0.00570000000001,0.));
#8789=CARTESIAN_POINT('',(-7.47034547479885E-19,0.00695,-0.0061));
#8790=CARTESIAN_POINT('Origin',(0.,0.,0.));
#8791=CARTESIAN_POINT('',(-7.22541611496938E-19,-0.00570000000001,-0.0059));
#8792=CARTESIAN_POINT('Origin',(0.,-0.00570000000001,0.));
#8793=CARTESIAN_POINT('',(-7.22541611496938E-19,0.,-0.0059));
#8794=CARTESIAN_POINT('Origin',(0.,-0.00695,0.));
#8795=CARTESIAN_POINT('',(7.71527483463054E-19,-0.00820000000001131,-0.00630000000000181));
#8796=CARTESIAN_POINT('',(7.47034547479885E-19,-0.00695,-0.0061));
#8797=CARTESIAN_POINT('Origin',(0.,-0.00820000000001,0.));
#8798=CARTESIAN_POINT('Origin',(0.,-0.0093500000782311,0.));
#8799=CARTESIAN_POINT('',(-7.71527483462833E-19,-0.0105000001564722,-0.0063));
#8800=CARTESIAN_POINT('Origin',(0.,-0.0105000001564722,0.));
#8801=CARTESIAN_POINT('',(-7.71527483462833E-19,-0.0093500000782311,-0.0063));
#8802=CARTESIAN_POINT('Origin',(0.,-0.0105000001564622,0.00700000010430813));
#8803=CARTESIAN_POINT('',(-8.57252772177209E-19,-0.0105000001564722,-0.00700000010430813));
#8804=CARTESIAN_POINT('Origin',(0.,-0.0105000001564722,0.));
#8805=CARTESIAN_POINT('Origin',(0.,-0.0107500001601875,0.));
#8806=CARTESIAN_POINT('',(-8.57252772177209E-19,-0.0110000001639228,-0.00700000010430813));
#8807=CARTESIAN_POINT('Origin',(0.,-0.0110000001639228,0.));
#8808=CARTESIAN_POINT('',(-8.57252772177209E-19,-0.0107500001601875,-0.00700000010430813));
#8809=CARTESIAN_POINT('Origin',(0.,-0.0110000001639128,0.0065));
#8810=CARTESIAN_POINT('Origin',(0.,-0.00875,0.00715));
#8811=CARTESIAN_POINT('',(-8.75622461390357E-19,-0.00875000000001,-0.00715));
#8812=CARTESIAN_POINT('Origin',(0.,-0.00875000000001,0.));
#8813=CARTESIAN_POINT('Origin',(0.,-0.0082,0.));
#8814=CARTESIAN_POINT('',(-8.75622461390357E-19,-0.00765000000001,-0.00715));
#8815=CARTESIAN_POINT('Origin',(0.,-0.00765000000001,0.));
#8816=CARTESIAN_POINT('',(-8.75622461390357E-19,-0.0082,-0.00715));
#8817=CARTESIAN_POINT('Origin',(0.,-0.00765,0.0075));
#8818=CARTESIAN_POINT('',(-9.18485099360515E-19,-0.00765000000001,-0.0075));
#8819=CARTESIAN_POINT('Origin',(0.,-0.00765000000001,0.));
#8820=CARTESIAN_POINT('Origin',(0.,0.,0.));
#8821=CARTESIAN_POINT('',(-9.18485099360515E-19,0.00765000000001,-0.0075));
#8822=CARTESIAN_POINT('Origin',(0.,0.00765000000001,0.));
#8823=CARTESIAN_POINT('',(-9.18485099360515E-19,0.,-0.0075));
#8824=CARTESIAN_POINT('Origin',(0.,0.00765,0.00715));
#8825=CARTESIAN_POINT('',(-8.75622461390357E-19,0.00765000000001,-0.00715));
#8826=CARTESIAN_POINT('Origin',(0.,0.00765000000001,0.));
#8827=CARTESIAN_POINT('Origin',(0.,0.0082,0.));
#8828=CARTESIAN_POINT('',(-8.75622461390357E-19,0.00875000000001,-0.00715));
#8829=CARTESIAN_POINT('Origin',(0.,0.00875000000001,0.));
#8830=CARTESIAN_POINT('',(-8.75622461390357E-19,0.0082,-0.00715));
#8831=CARTESIAN_POINT('Origin',(0.,0.00875,0.0075));
#8928=UNCERTAINTY_MEASURE_WITH_UNIT(LENGTH_MEASURE(1.E-5),#8945,
'DISTANCE_ACCURACY_VALUE',
'Maximum model space distance between geometric entities at asserted c
onnectivities');
#8932=UNCERTAINTY_MEASURE_WITH_UNIT(LENGTH_MEASURE(1.E-5),#8945,
'DISTANCE_ACCURACY_VALUE',
'Maximum model space distance between geometric entities at asserted c
onnectivities');
#8940=(
GEOMETRIC_REPRESENTATION_CONTEXT(3)
GLOBAL_UNCERTAINTY_ASSIGNED_CONTEXT((#8928))
GLOBAL_UNIT_ASSIGNED_CONTEXT((#8945,#8946,#8947))
REPRESENTATION_CONTEXT('','3D')
);
#8944=(
GEOMETRIC_REPRESENTATION_CONTEXT(3)
GLOBAL_UNCERTAINTY_ASSIGNED_CONTEXT((#8932))
GLOBAL_UNIT_ASSIGNED_CONTEXT((#8945,#8946,#8947))
REPRESENTATION_CONTEXT('','3D')
);
#8945=(
LENGTH_UNIT()
NAMED_UNIT(*)
SI_UNIT($,.METRE.)
);
#8946=(
NAMED_UNIT(*)
PLANE_ANGLE_UNIT()
SI_UNIT($,.RADIAN.)
);
#8947=(
NAMED_UNIT(*)
SI_UNIT($,.STERADIAN.)
SOLID_ANGLE_UNIT()
);
#8955=SHAPE_DEFINITION_REPRESENTATION(#8966,#8999);
#8966=PRODUCT_DEFINITION_SHAPE('',$,#9011);
#8999=SHAPE_REPRESENTATION('',(#5695),#8940);
#9003=PRODUCT_DEFINITION_CONTEXT('part definition',#9038,'design');
#9011=PRODUCT_DEFINITION('Ball Bushing','Ball Bushing',#9022,#9003);
#9022=PRODUCT_DEFINITION_FORMATION('',$,#9047);
#9038=APPLICATION_CONTEXT('Managed model based 3d engineering');
#9039=PRODUCT_CONTEXT('part definition',#9038,'mechanical');
#9047=PRODUCT('Ball Bushing','Ball Bushing',
'LEGAL AND USAGE DISCLAIMER: this Data/Model is provided \X2\201C\X0\A
S IS\X2\201D\X0\ for informational and representational only. It is a 
geometric approximation and is NOT engineered, certified, or guarantee
d for dimensional accuracy, exact tolerances, or production-level prec
ision. Vendor disclaims all implied warranties including fitness for a
 particular purpose. DO NOT USE FOR DIRECT PHYSICAL MANUFACTURING, AUT
OMATED PRODUCTION, OR SAFETY-CRITICAL SYSTEMS without independent engi
neering verification and resolution of any design discrepancies.',(#9039));
#9054=PRESENTATION_STYLE_ASSIGNMENT((#9059));
#9059=SURFACE_STYLE_USAGE(.BOTH.,#9064);
#9064=SURFACE_SIDE_STYLE('',(#9069));
#9069=SURFACE_STYLE_FILL_AREA(#9074);
#9074=FILL_AREA_STYLE('Opaque(137,137,137)',(#9079));
#9079=FILL_AREA_STYLE_COLOUR('Opaque(137,137,137)',#9084);
#9084=COLOUR_RGB('Opaque(137,137,137)',0.537254901960784,0.537254901960784,
0.537254901960784);
ENDSEC;
END-ISO-10303-21;
